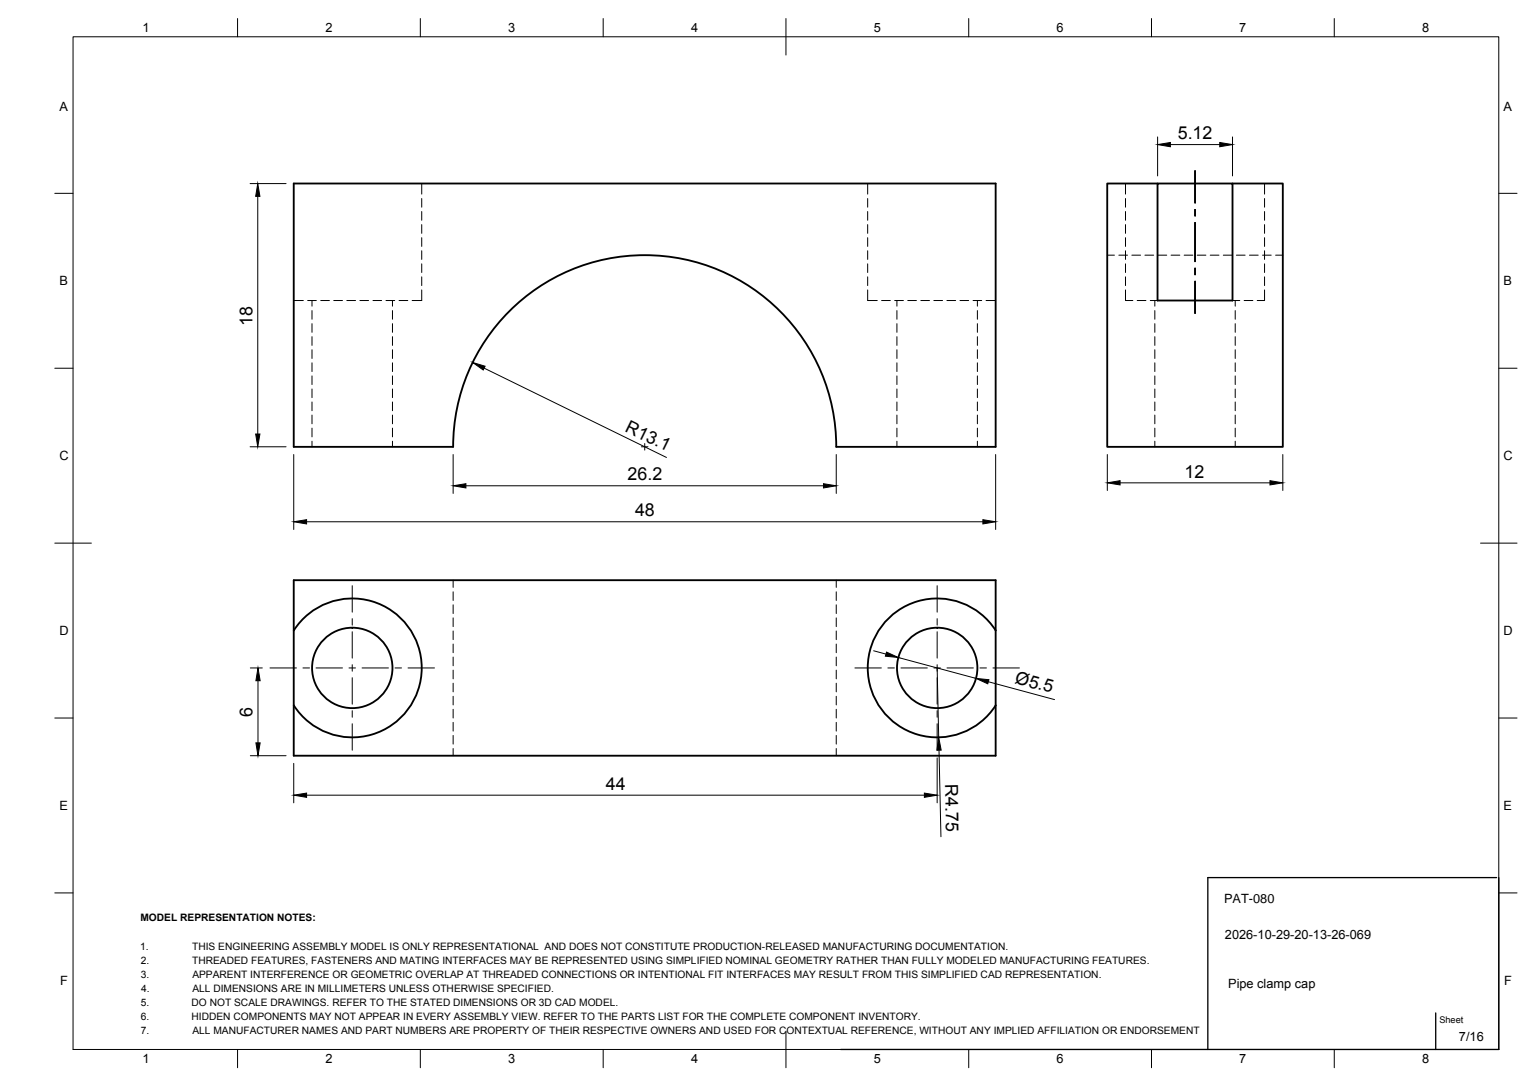
ISO-10303-21;
HEADER;
/* Generated by software containing ST-Developer
 * from STEP Tools, Inc. (www.steptools.com) 
 */

FILE_DESCRIPTION(
/* description */ ('PAT-080'),
/* implementation_level */ '2;1');

FILE_NAME(
/* name */ 'Pipe clamp cap.step',
/* time_stamp */ '2026-10-29T20:13:47-07:00',
/* author */ (''),
/* organization */ (''),
/* preprocessor_version */ 'ST-DEVELOPER v20.2',
/* originating_system */ 'Autodesk Translation Framework v15.17.0.0',
/* authorisation */ '');

FILE_SCHEMA (('AUTOMOTIVE_DESIGN { 1 0 10303 214 3 1 1 }'));
ENDSEC;

DATA;
#10=MECHANICAL_DESIGN_GEOMETRIC_PRESENTATION_REPRESENTATION('',(#250),#6878);
#212=SHAPE_REPRESENTATION_RELATIONSHIP('SRR','None',#6968,#231);
#231=ADVANCED_BREP_SHAPE_REPRESENTATION('',(#269),#6863);
#250=STYLED_ITEM('',(#7143),#269);
#269=MANIFOLD_SOLID_BREP('Body1',#3866);
#295=FACE_BOUND('',#785,.T.);
#296=FACE_BOUND('',#788,.T.);
#297=FACE_BOUND('',#797,.T.);
#298=FACE_BOUND('',#801,.T.);
#392=PLANE('',#4162);
#393=PLANE('',#4167);
#394=PLANE('',#4172);
#395=PLANE('',#4173);
#396=PLANE('',#4181);
#397=PLANE('',#4182);
#398=PLANE('',#4183);
#399=PLANE('',#4184);
#400=PLANE('',#4185);
#544=FACE_OUTER_BOUND('',#784,.T.);
#545=FACE_OUTER_BOUND('',#786,.T.);
#546=FACE_OUTER_BOUND('',#787,.T.);
#547=FACE_OUTER_BOUND('',#789,.T.);
#548=FACE_OUTER_BOUND('',#790,.T.);
#549=FACE_OUTER_BOUND('',#791,.T.);
#550=FACE_OUTER_BOUND('',#792,.T.);
#551=FACE_OUTER_BOUND('',#793,.T.);
#552=FACE_OUTER_BOUND('',#794,.T.);
#553=FACE_OUTER_BOUND('',#795,.T.);
#554=FACE_OUTER_BOUND('',#796,.T.);
#555=FACE_OUTER_BOUND('',#798,.T.);
#556=FACE_OUTER_BOUND('',#799,.T.);
#557=FACE_OUTER_BOUND('',#800,.T.);
#784=EDGE_LOOP('',(#2812,#2813));
#785=EDGE_LOOP('',(#2814));
#786=EDGE_LOOP('',(#2815,#2816,#2817,#2818));
#787=EDGE_LOOP('',(#2819,#2820));
#788=EDGE_LOOP('',(#2821));
#789=EDGE_LOOP('',(#2822,#2823,#2824,#2825));
#790=EDGE_LOOP('',(#2826,#2827,#2828,#2829,#2830,#2831,#2832,#2833));
#791=EDGE_LOOP('',(#2834,#2835,#2836,#2837,#2838,#2839,#2840,#2841));
#792=EDGE_LOOP('',(#2842,#2843,#2844,#2845));
#793=EDGE_LOOP('',(#2846,#2847,#2848,#2849));
#794=EDGE_LOOP('',(#2850,#2851,#2852,#2853));
#795=EDGE_LOOP('',(#2854,#2855,#2856,#2857,#2858,#2859));
#796=EDGE_LOOP('',(#2860,#2861,#2862,#2863));
#797=EDGE_LOOP('',(#2864));
#798=EDGE_LOOP('',(#2865,#2866,#2867,#2868,#2869,#2870));
#799=EDGE_LOOP('',(#2871,#2872,#2873,#2874,#2875,#2876,#2877,#2878));
#800=EDGE_LOOP('',(#2879,#2880,#2881,#2882));
#801=EDGE_LOOP('',(#2883));
#1112=LINE('',#5952,#1427);
#1113=LINE('',#5958,#1428);
#1114=LINE('',#5961,#1429);
#1115=LINE('',#5965,#1430);
#1116=LINE('',#5971,#1431);
#1117=LINE('',#5974,#1432);
#1118=LINE('',#5977,#1433);
#1119=LINE('',#5979,#1434);
#1120=LINE('',#5981,#1435);
#1121=LINE('',#5983,#1436);
#1122=LINE('',#5984,#1437);
#1123=LINE('',#5987,#1438);
#1124=LINE('',#5989,#1439);
#1125=LINE('',#5991,#1440);
#1126=LINE('',#5993,#1441);
#1127=LINE('',#5994,#1442);
#1128=LINE('',#5998,#1443);
#1129=LINE('',#6002,#1444);
#1130=LINE('',#6008,#1445);
#1131=LINE('',#6011,#1446);
#1132=LINE('',#6013,#1447);
#1133=LINE('',#6014,#1448);
#1134=LINE('',#6015,#1449);
#1135=LINE('',#6017,#1450);
#1136=LINE('',#6019,#1451);
#1137=LINE('',#6020,#1452);
#1427=VECTOR('',#4756,1.);
#1428=VECTOR('',#4763,1.);
#1429=VECTOR('',#4766,1.);
#1430=VECTOR('',#4769,1.);
#1431=VECTOR('',#4776,1.);
#1432=VECTOR('',#4779,1.);
#1433=VECTOR('',#4782,1.);
#1434=VECTOR('',#4783,1.);
#1435=VECTOR('',#4784,1.);
#1436=VECTOR('',#4785,1.);
#1437=VECTOR('',#4786,1.);
#1438=VECTOR('',#4789,1.);
#1439=VECTOR('',#4790,1.);
#1440=VECTOR('',#4791,1.);
#1441=VECTOR('',#4792,1.);
#1442=VECTOR('',#4793,1.);
#1443=VECTOR('',#4798,0.275);
#1444=VECTOR('',#4803,0.275);
#1445=VECTOR('',#4808,1.);
#1446=VECTOR('',#4811,1.);
#1447=VECTOR('',#4814,1.);
#1448=VECTOR('',#4815,1.);
#1449=VECTOR('',#4816,1.);
#1450=VECTOR('',#4819,1.);
#1451=VECTOR('',#4822,1.);
#1452=VECTOR('',#4823,1.);
#1676=CIRCLE('',#4163,0.475);
#1677=CIRCLE('',#4164,0.275);
#1678=CIRCLE('',#4166,0.475);
#1679=CIRCLE('',#4168,0.475);
#1680=CIRCLE('',#4169,0.275);
#1681=CIRCLE('',#4171,0.475);
#1682=CIRCLE('',#4175,0.275);
#1683=CIRCLE('',#4177,0.275);
#1684=CIRCLE('',#4179,1.31);
#1685=CIRCLE('',#4180,1.31);
#1878=VERTEX_POINT('',#5950);
#1879=VERTEX_POINT('',#5951);
#1880=VERTEX_POINT('',#5954);
#1881=VERTEX_POINT('',#5957);
#1882=VERTEX_POINT('',#5959);
#1883=VERTEX_POINT('',#5963);
#1884=VERTEX_POINT('',#5964);
#1885=VERTEX_POINT('',#5967);
#1886=VERTEX_POINT('',#5970);
#1887=VERTEX_POINT('',#5972);
#1888=VERTEX_POINT('',#5976);
#1889=VERTEX_POINT('',#5978);
#1890=VERTEX_POINT('',#5980);
#1891=VERTEX_POINT('',#5982);
#1892=VERTEX_POINT('',#5986);
#1893=VERTEX_POINT('',#5988);
#1894=VERTEX_POINT('',#5990);
#1895=VERTEX_POINT('',#5992);
#1896=VERTEX_POINT('',#5996);
#1897=VERTEX_POINT('',#6000);
#1898=VERTEX_POINT('',#6004);
#1899=VERTEX_POINT('',#6005);
#1900=VERTEX_POINT('',#6007);
#1901=VERTEX_POINT('',#6009);
#2229=EDGE_CURVE('',#1878,#1879,#1112,.T.);
#2230=EDGE_CURVE('',#1878,#1879,#1676,.T.);
#2231=EDGE_CURVE('',#1880,#1880,#1677,.T.);
#2232=EDGE_CURVE('',#1881,#1878,#1113,.T.);
#2233=EDGE_CURVE('',#1882,#1881,#1678,.T.);
#2234=EDGE_CURVE('',#1879,#1882,#1114,.T.);
#2235=EDGE_CURVE('',#1883,#1884,#1115,.T.);
#2236=EDGE_CURVE('',#1883,#1884,#1679,.T.);
#2237=EDGE_CURVE('',#1885,#1885,#1680,.T.);
#2238=EDGE_CURVE('',#1886,#1883,#1116,.T.);
#2239=EDGE_CURVE('',#1887,#1886,#1681,.T.);
#2240=EDGE_CURVE('',#1884,#1887,#1117,.T.);
#2241=EDGE_CURVE('',#1888,#1882,#1118,.T.);
#2242=EDGE_CURVE('',#1889,#1888,#1119,.T.);
#2243=EDGE_CURVE('',#1889,#1890,#1120,.T.);
#2244=EDGE_CURVE('',#1890,#1891,#1121,.T.);
#2245=EDGE_CURVE('',#1881,#1891,#1122,.T.);
#2246=EDGE_CURVE('',#1892,#1887,#1123,.T.);
#2247=EDGE_CURVE('',#1893,#1892,#1124,.T.);
#2248=EDGE_CURVE('',#1893,#1894,#1125,.T.);
#2249=EDGE_CURVE('',#1894,#1895,#1126,.T.);
#2250=EDGE_CURVE('',#1886,#1895,#1127,.T.);
#2251=EDGE_CURVE('',#1896,#1896,#1682,.T.);
#2252=EDGE_CURVE('',#1896,#1880,#1128,.T.);
#2253=EDGE_CURVE('',#1897,#1897,#1683,.T.);
#2254=EDGE_CURVE('',#1897,#1885,#1129,.T.);
#2255=EDGE_CURVE('',#1898,#1899,#1684,.T.);
#2256=EDGE_CURVE('',#1900,#1898,#1130,.T.);
#2257=EDGE_CURVE('',#1901,#1900,#1685,.T.);
#2258=EDGE_CURVE('',#1899,#1901,#1131,.T.);
#2259=EDGE_CURVE('',#1900,#1893,#1132,.T.);
#2260=EDGE_CURVE('',#1891,#1892,#1133,.T.);
#2261=EDGE_CURVE('',#1890,#1901,#1134,.T.);
#2262=EDGE_CURVE('',#1894,#1898,#1135,.T.);
#2263=EDGE_CURVE('',#1899,#1889,#1136,.T.);
#2264=EDGE_CURVE('',#1895,#1888,#1137,.T.);
#2812=ORIENTED_EDGE('',*,*,#2229,.F.);
#2813=ORIENTED_EDGE('',*,*,#2230,.T.);
#2814=ORIENTED_EDGE('',*,*,#2231,.F.);
#2815=ORIENTED_EDGE('',*,*,#2232,.F.);
#2816=ORIENTED_EDGE('',*,*,#2233,.F.);
#2817=ORIENTED_EDGE('',*,*,#2234,.F.);
#2818=ORIENTED_EDGE('',*,*,#2230,.F.);
#2819=ORIENTED_EDGE('',*,*,#2235,.F.);
#2820=ORIENTED_EDGE('',*,*,#2236,.T.);
#2821=ORIENTED_EDGE('',*,*,#2237,.F.);
#2822=ORIENTED_EDGE('',*,*,#2238,.F.);
#2823=ORIENTED_EDGE('',*,*,#2239,.F.);
#2824=ORIENTED_EDGE('',*,*,#2240,.F.);
#2825=ORIENTED_EDGE('',*,*,#2236,.F.);
#2826=ORIENTED_EDGE('',*,*,#2232,.T.);
#2827=ORIENTED_EDGE('',*,*,#2229,.T.);
#2828=ORIENTED_EDGE('',*,*,#2234,.T.);
#2829=ORIENTED_EDGE('',*,*,#2241,.F.);
#2830=ORIENTED_EDGE('',*,*,#2242,.F.);
#2831=ORIENTED_EDGE('',*,*,#2243,.T.);
#2832=ORIENTED_EDGE('',*,*,#2244,.T.);
#2833=ORIENTED_EDGE('',*,*,#2245,.F.);
#2834=ORIENTED_EDGE('',*,*,#2238,.T.);
#2835=ORIENTED_EDGE('',*,*,#2235,.T.);
#2836=ORIENTED_EDGE('',*,*,#2240,.T.);
#2837=ORIENTED_EDGE('',*,*,#2246,.F.);
#2838=ORIENTED_EDGE('',*,*,#2247,.F.);
#2839=ORIENTED_EDGE('',*,*,#2248,.T.);
#2840=ORIENTED_EDGE('',*,*,#2249,.T.);
#2841=ORIENTED_EDGE('',*,*,#2250,.F.);
#2842=ORIENTED_EDGE('',*,*,#2251,.F.);
#2843=ORIENTED_EDGE('',*,*,#2252,.T.);
#2844=ORIENTED_EDGE('',*,*,#2231,.T.);
#2845=ORIENTED_EDGE('',*,*,#2252,.F.);
#2846=ORIENTED_EDGE('',*,*,#2253,.F.);
#2847=ORIENTED_EDGE('',*,*,#2254,.T.);
#2848=ORIENTED_EDGE('',*,*,#2237,.T.);
#2849=ORIENTED_EDGE('',*,*,#2254,.F.);
#2850=ORIENTED_EDGE('',*,*,#2255,.F.);
#2851=ORIENTED_EDGE('',*,*,#2256,.F.);
#2852=ORIENTED_EDGE('',*,*,#2257,.F.);
#2853=ORIENTED_EDGE('',*,*,#2258,.F.);
#2854=ORIENTED_EDGE('',*,*,#2257,.T.);
#2855=ORIENTED_EDGE('',*,*,#2259,.T.);
#2856=ORIENTED_EDGE('',*,*,#2247,.T.);
#2857=ORIENTED_EDGE('',*,*,#2260,.F.);
#2858=ORIENTED_EDGE('',*,*,#2244,.F.);
#2859=ORIENTED_EDGE('',*,*,#2261,.T.);
#2860=ORIENTED_EDGE('',*,*,#2256,.T.);
#2861=ORIENTED_EDGE('',*,*,#2262,.F.);
#2862=ORIENTED_EDGE('',*,*,#2248,.F.);
#2863=ORIENTED_EDGE('',*,*,#2259,.F.);
#2864=ORIENTED_EDGE('',*,*,#2253,.T.);
#2865=ORIENTED_EDGE('',*,*,#2255,.T.);
#2866=ORIENTED_EDGE('',*,*,#2263,.T.);
#2867=ORIENTED_EDGE('',*,*,#2242,.T.);
#2868=ORIENTED_EDGE('',*,*,#2264,.F.);
#2869=ORIENTED_EDGE('',*,*,#2249,.F.);
#2870=ORIENTED_EDGE('',*,*,#2262,.T.);
#2871=ORIENTED_EDGE('',*,*,#2233,.T.);
#2872=ORIENTED_EDGE('',*,*,#2245,.T.);
#2873=ORIENTED_EDGE('',*,*,#2260,.T.);
#2874=ORIENTED_EDGE('',*,*,#2246,.T.);
#2875=ORIENTED_EDGE('',*,*,#2239,.T.);
#2876=ORIENTED_EDGE('',*,*,#2250,.T.);
#2877=ORIENTED_EDGE('',*,*,#2264,.T.);
#2878=ORIENTED_EDGE('',*,*,#2241,.T.);
#2879=ORIENTED_EDGE('',*,*,#2258,.T.);
#2880=ORIENTED_EDGE('',*,*,#2261,.F.);
#2881=ORIENTED_EDGE('',*,*,#2243,.F.);
#2882=ORIENTED_EDGE('',*,*,#2263,.F.);
#2883=ORIENTED_EDGE('',*,*,#2251,.T.);
#3579=CYLINDRICAL_SURFACE('',#4165,0.475);
#3580=CYLINDRICAL_SURFACE('',#4170,0.475);
#3581=CYLINDRICAL_SURFACE('',#4174,0.275);
#3582=CYLINDRICAL_SURFACE('',#4176,0.275);
#3583=CYLINDRICAL_SURFACE('',#4178,1.31);
#3680=ADVANCED_FACE('',(#544,#295),#392,.T.);
#3681=ADVANCED_FACE('',(#545),#3579,.F.);
#3682=ADVANCED_FACE('',(#546,#296),#393,.T.);
#3683=ADVANCED_FACE('',(#547),#3580,.F.);
#3684=ADVANCED_FACE('',(#548),#394,.T.);
#3685=ADVANCED_FACE('',(#549),#395,.T.);
#3686=ADVANCED_FACE('',(#550),#3581,.F.);
#3687=ADVANCED_FACE('',(#551),#3582,.F.);
#3688=ADVANCED_FACE('',(#552),#3583,.F.);
#3689=ADVANCED_FACE('',(#553),#396,.T.);
#3690=ADVANCED_FACE('',(#554,#297),#397,.F.);
#3691=ADVANCED_FACE('',(#555),#398,.T.);
#3692=ADVANCED_FACE('',(#556),#399,.T.);
#3693=ADVANCED_FACE('',(#557,#298),#400,.F.);
#3866=CLOSED_SHELL('',(#3680,#3681,#3682,#3683,#3684,#3685,#3686,#3687,
#3688,#3689,#3690,#3691,#3692,#3693));
#4161=AXIS2_PLACEMENT_3D('',#5948,#4752,#4753);
#4162=AXIS2_PLACEMENT_3D('',#5949,#4754,#4755);
#4163=AXIS2_PLACEMENT_3D('',#5953,#4757,#4758);
#4164=AXIS2_PLACEMENT_3D('',#5955,#4759,#4760);
#4165=AXIS2_PLACEMENT_3D('',#5956,#4761,#4762);
#4166=AXIS2_PLACEMENT_3D('',#5960,#4764,#4765);
#4167=AXIS2_PLACEMENT_3D('',#5962,#4767,#4768);
#4168=AXIS2_PLACEMENT_3D('',#5966,#4770,#4771);
#4169=AXIS2_PLACEMENT_3D('',#5968,#4772,#4773);
#4170=AXIS2_PLACEMENT_3D('',#5969,#4774,#4775);
#4171=AXIS2_PLACEMENT_3D('',#5973,#4777,#4778);
#4172=AXIS2_PLACEMENT_3D('',#5975,#4780,#4781);
#4173=AXIS2_PLACEMENT_3D('',#5985,#4787,#4788);
#4174=AXIS2_PLACEMENT_3D('',#5995,#4794,#4795);
#4175=AXIS2_PLACEMENT_3D('',#5997,#4796,#4797);
#4176=AXIS2_PLACEMENT_3D('',#5999,#4799,#4800);
#4177=AXIS2_PLACEMENT_3D('',#6001,#4801,#4802);
#4178=AXIS2_PLACEMENT_3D('',#6003,#4804,#4805);
#4179=AXIS2_PLACEMENT_3D('',#6006,#4806,#4807);
#4180=AXIS2_PLACEMENT_3D('',#6010,#4809,#4810);
#4181=AXIS2_PLACEMENT_3D('',#6012,#4812,#4813);
#4182=AXIS2_PLACEMENT_3D('',#6016,#4817,#4818);
#4183=AXIS2_PLACEMENT_3D('',#6018,#4820,#4821);
#4184=AXIS2_PLACEMENT_3D('',#6021,#4824,#4825);
#4185=AXIS2_PLACEMENT_3D('',#6022,#4826,#4827);
#4752=DIRECTION('axis',(0.,0.,1.));
#4753=DIRECTION('refdir',(1.,0.,0.));
#4754=DIRECTION('center_axis',(0.,0.,1.));
#4755=DIRECTION('ref_axis',(1.,0.,0.));
#4756=DIRECTION('',(-1.,0.,0.));
#4757=DIRECTION('center_axis',(0.,0.,1.));
#4758=DIRECTION('ref_axis',(1.,0.,0.));
#4759=DIRECTION('center_axis',(0.,0.,1.));
#4760=DIRECTION('ref_axis',(1.,0.,0.));
#4761=DIRECTION('center_axis',(0.,0.,1.));
#4762=DIRECTION('ref_axis',(6.12323399573677E-17,1.,0.));
#4763=DIRECTION('',(0.,0.,-1.));
#4764=DIRECTION('center_axis',(0.,0.,-1.));
#4765=DIRECTION('ref_axis',(1.,0.,0.));
#4766=DIRECTION('',(0.,0.,1.));
#4767=DIRECTION('center_axis',(0.,0.,1.));
#4768=DIRECTION('ref_axis',(1.,0.,0.));
#4769=DIRECTION('',(1.,0.,0.));
#4770=DIRECTION('center_axis',(0.,0.,1.));
#4771=DIRECTION('ref_axis',(1.,0.,0.));
#4772=DIRECTION('center_axis',(0.,0.,1.));
#4773=DIRECTION('ref_axis',(1.,0.,0.));
#4774=DIRECTION('center_axis',(0.,0.,1.));
#4775=DIRECTION('ref_axis',(-1.83697019872103E-16,-1.,0.));
#4776=DIRECTION('',(0.,0.,-1.));
#4777=DIRECTION('center_axis',(0.,0.,-1.));
#4778=DIRECTION('ref_axis',(1.,0.,0.));
#4779=DIRECTION('',(0.,0.,1.));
#4780=DIRECTION('center_axis',(0.,-1.,0.));
#4781=DIRECTION('ref_axis',(1.,0.,0.));
#4782=DIRECTION('',(1.,0.,0.));
#4783=DIRECTION('',(0.,0.,1.));
#4784=DIRECTION('',(1.,0.,0.));
#4785=DIRECTION('',(0.,0.,1.));
#4786=DIRECTION('',(1.,0.,0.));
#4787=DIRECTION('center_axis',(0.,1.,0.));
#4788=DIRECTION('ref_axis',(-1.,0.,0.));
#4789=DIRECTION('',(-1.,0.,0.));
#4790=DIRECTION('',(0.,0.,1.));
#4791=DIRECTION('',(-1.,0.,0.));
#4792=DIRECTION('',(0.,0.,1.));
#4793=DIRECTION('',(-1.,0.,0.));
#4794=DIRECTION('center_axis',(0.,0.,1.));
#4795=DIRECTION('ref_axis',(1.,0.,0.));
#4796=DIRECTION('center_axis',(0.,0.,1.));
#4797=DIRECTION('ref_axis',(1.,0.,0.));
#4798=DIRECTION('',(0.,0.,1.));
#4799=DIRECTION('center_axis',(0.,0.,1.));
#4800=DIRECTION('ref_axis',(1.,0.,0.));
#4801=DIRECTION('center_axis',(0.,0.,1.));
#4802=DIRECTION('ref_axis',(1.,0.,0.));
#4803=DIRECTION('',(0.,0.,1.));
#4804=DIRECTION('center_axis',(1.,0.,0.));
#4805=DIRECTION('ref_axis',(0.,1.22464679914735E-16,1.));
#4806=DIRECTION('center_axis',(1.,0.,0.));
#4807=DIRECTION('ref_axis',(0.,0.,-1.));
#4808=DIRECTION('',(-1.,0.,0.));
#4809=DIRECTION('center_axis',(-1.,0.,0.));
#4810=DIRECTION('ref_axis',(0.,0.,-1.));
#4811=DIRECTION('',(1.,0.,0.));
#4812=DIRECTION('center_axis',(1.,0.,0.));
#4813=DIRECTION('ref_axis',(0.,1.,0.));
#4814=DIRECTION('',(0.,1.,0.));
#4815=DIRECTION('',(0.,1.,0.));
#4816=DIRECTION('',(0.,1.,0.));
#4817=DIRECTION('center_axis',(0.,0.,1.));
#4818=DIRECTION('ref_axis',(1.,0.,0.));
#4819=DIRECTION('',(0.,-1.,0.));
#4820=DIRECTION('center_axis',(-1.,0.,0.));
#4821=DIRECTION('ref_axis',(0.,-1.,0.));
#4822=DIRECTION('',(0.,-1.,0.));
#4823=DIRECTION('',(0.,-1.,0.));
#4824=DIRECTION('center_axis',(0.,0.,1.));
#4825=DIRECTION('ref_axis',(1.,0.,0.));
#4826=DIRECTION('center_axis',(0.,0.,1.));
#4827=DIRECTION('ref_axis',(1.,0.,0.));
#5948=CARTESIAN_POINT('',(0.,0.,0.));
#5949=CARTESIAN_POINT('Origin',(-4.5,-2.,7.));
#5950=CARTESIAN_POINT('',(-4.24382623085101,-2.4,7.));
#5951=CARTESIAN_POINT('',(-4.75617376914899,-2.4,7.));
#5952=CARTESIAN_POINT('',(-4.8,-2.4,7.));
#5953=CARTESIAN_POINT('Origin',(-4.5,-2.,7.));
#5954=CARTESIAN_POINT('',(-4.775,-2.,7.));
#5955=CARTESIAN_POINT('Origin',(-4.5,-2.,7.));
#5956=CARTESIAN_POINT('Origin',(-4.5,-2.,7.));
#5957=CARTESIAN_POINT('',(-4.24382623085101,-2.4,7.8));
#5958=CARTESIAN_POINT('',(-4.24382623085101,-2.4,7.));
#5959=CARTESIAN_POINT('',(-4.75617376914899,-2.4,7.8));
#5960=CARTESIAN_POINT('Origin',(-4.5,-2.,7.8));
#5961=CARTESIAN_POINT('',(-4.75617376914899,-2.4,7.));
#5962=CARTESIAN_POINT('Origin',(-4.5,2.,7.));
#5963=CARTESIAN_POINT('',(-4.75617376914899,2.4,7.));
#5964=CARTESIAN_POINT('',(-4.24382623085101,2.4,7.));
#5965=CARTESIAN_POINT('',(-4.2,2.4,7.));
#5966=CARTESIAN_POINT('Origin',(-4.5,2.,7.));
#5967=CARTESIAN_POINT('',(-4.775,2.,7.));
#5968=CARTESIAN_POINT('Origin',(-4.5,2.,7.));
#5969=CARTESIAN_POINT('Origin',(-4.5,2.,7.));
#5970=CARTESIAN_POINT('',(-4.75617376914899,2.4,7.8));
#5971=CARTESIAN_POINT('',(-4.75617376914899,2.4,7.));
#5972=CARTESIAN_POINT('',(-4.24382623085101,2.4,7.8));
#5973=CARTESIAN_POINT('Origin',(-4.5,2.,7.8));
#5974=CARTESIAN_POINT('',(-4.24382623085101,2.4,7.));
#5975=CARTESIAN_POINT('Origin',(-5.1,-2.4,6.));
#5976=CARTESIAN_POINT('',(-5.1,-2.4,7.8));
#5977=CARTESIAN_POINT('',(-5.1,-2.4,7.8));
#5978=CARTESIAN_POINT('',(-5.1,-2.4,6.));
#5979=CARTESIAN_POINT('',(-5.1,-2.4,6.));
#5980=CARTESIAN_POINT('',(-3.9,-2.4,6.));
#5981=CARTESIAN_POINT('',(-5.1,-2.4,6.));
#5982=CARTESIAN_POINT('',(-3.9,-2.4,7.8));
#5983=CARTESIAN_POINT('',(-3.9,-2.4,6.));
#5984=CARTESIAN_POINT('',(-5.1,-2.4,7.8));
#5985=CARTESIAN_POINT('Origin',(-3.9,2.4,6.));
#5986=CARTESIAN_POINT('',(-3.9,2.4,7.8));
#5987=CARTESIAN_POINT('',(-3.9,2.4,7.8));
#5988=CARTESIAN_POINT('',(-3.9,2.4,6.));
#5989=CARTESIAN_POINT('',(-3.9,2.4,6.));
#5990=CARTESIAN_POINT('',(-5.1,2.4,6.));
#5991=CARTESIAN_POINT('',(-3.9,2.4,6.));
#5992=CARTESIAN_POINT('',(-5.1,2.4,7.8));
#5993=CARTESIAN_POINT('',(-5.1,2.4,6.));
#5994=CARTESIAN_POINT('',(-3.9,2.4,7.8));
#5995=CARTESIAN_POINT('Origin',(-4.5,-2.,5.9));
#5996=CARTESIAN_POINT('',(-4.775,-2.,6.));
#5997=CARTESIAN_POINT('Origin',(-4.5,-2.,6.));
#5998=CARTESIAN_POINT('',(-4.775,-2.,5.9));
#5999=CARTESIAN_POINT('Origin',(-4.5,2.,5.9));
#6000=CARTESIAN_POINT('',(-4.775,2.,6.));
#6001=CARTESIAN_POINT('Origin',(-4.5,2.,6.));
#6002=CARTESIAN_POINT('',(-4.775,2.,5.9));
#6003=CARTESIAN_POINT('Origin',(-5.2,0.,6.));
#6004=CARTESIAN_POINT('',(-5.1,1.31,6.));
#6005=CARTESIAN_POINT('',(-5.1,-1.31,6.));
#6006=CARTESIAN_POINT('Origin',(-5.1,0.,6.));
#6007=CARTESIAN_POINT('',(-3.9,1.31,6.));
#6008=CARTESIAN_POINT('',(-5.2,1.31,6.));
#6009=CARTESIAN_POINT('',(-3.9,-1.31,6.));
#6010=CARTESIAN_POINT('Origin',(-3.9,0.,6.));
#6011=CARTESIAN_POINT('',(-5.2,-1.31,6.));
#6012=CARTESIAN_POINT('Origin',(-3.9,-2.4,6.));
#6013=CARTESIAN_POINT('',(-3.9,-2.4,6.));
#6014=CARTESIAN_POINT('',(-3.9,-2.4,7.8));
#6015=CARTESIAN_POINT('',(-3.9,-2.4,6.));
#6016=CARTESIAN_POINT('Origin',(-4.5,0.,6.));
#6017=CARTESIAN_POINT('',(-5.1,2.4,6.));
#6018=CARTESIAN_POINT('Origin',(-5.1,2.4,6.));
#6019=CARTESIAN_POINT('',(-5.1,2.4,6.));
#6020=CARTESIAN_POINT('',(-5.1,2.4,7.8));
#6021=CARTESIAN_POINT('Origin',(-4.5,0.,7.8));
#6022=CARTESIAN_POINT('Origin',(-4.5,0.,6.));
#6842=UNCERTAINTY_MEASURE_WITH_UNIT(LENGTH_MEASURE(0.001),#6879,
'DISTANCE_ACCURACY_VALUE',
'Maximum model space distance between geometric entities at asserted c
onnectivities');
#6857=UNCERTAINTY_MEASURE_WITH_UNIT(LENGTH_MEASURE(0.001),#6879,
'DISTANCE_ACCURACY_VALUE',
'Maximum model space distance between geometric entities at asserted c
onnectivities');
#6863=(
GEOMETRIC_REPRESENTATION_CONTEXT(3)
GLOBAL_UNCERTAINTY_ASSIGNED_CONTEXT((#6842))
GLOBAL_UNIT_ASSIGNED_CONTEXT((#6879,#6881,#6882))
REPRESENTATION_CONTEXT('','3D')
);
#6878=(
GEOMETRIC_REPRESENTATION_CONTEXT(3)
GLOBAL_UNCERTAINTY_ASSIGNED_CONTEXT((#6857))
GLOBAL_UNIT_ASSIGNED_CONTEXT((#6879,#6881,#6882))
REPRESENTATION_CONTEXT('','3D')
);
#6879=(
LENGTH_UNIT()
NAMED_UNIT(*)
SI_UNIT(.CENTI.,.METRE.)
);
#6881=(
NAMED_UNIT(*)
PLANE_ANGLE_UNIT()
SI_UNIT($,.RADIAN.)
);
#6882=(
NAMED_UNIT(*)
SI_UNIT($,.STERADIAN.)
SOLID_ANGLE_UNIT()
);
#6888=SHAPE_DEFINITION_REPRESENTATION(#6908,#6968);
#6908=PRODUCT_DEFINITION_SHAPE('',$,#6989);
#6968=SHAPE_REPRESENTATION('',(#4161),#6863);
#6983=PRODUCT_DEFINITION_CONTEXT('part definition',#7045,'design');
#6989=PRODUCT_DEFINITION('Pipe clamp cap','Pipe clamp cap',#7009,
#6983);
#7009=PRODUCT_DEFINITION_FORMATION('',$,#7052);
#7045=APPLICATION_CONTEXT(
'Core Data for Automotive Mechanical Design Process');
#7046=PRODUCT_CONTEXT('part definition',#7045,'mechanical');
#7052=PRODUCT('Pipe clamp cap','Pipe clamp cap',
'Pipe clamp cap',(#7046));
#7137=COLOUR_RGB('Off White',0.89,0.88,0.83);
#7138=FILL_AREA_STYLE_COLOUR('',#7137);
#7139=FILL_AREA_STYLE('',(#7138));
#7140=SURFACE_STYLE_FILL_AREA(#7139);
#7141=SURFACE_SIDE_STYLE('',(#7140));
#7142=SURFACE_STYLE_USAGE(.BOTH.,#7141);
#7143=PRESENTATION_STYLE_ASSIGNMENT((#7142));
ENDSEC;
END-ISO-10303-21;
